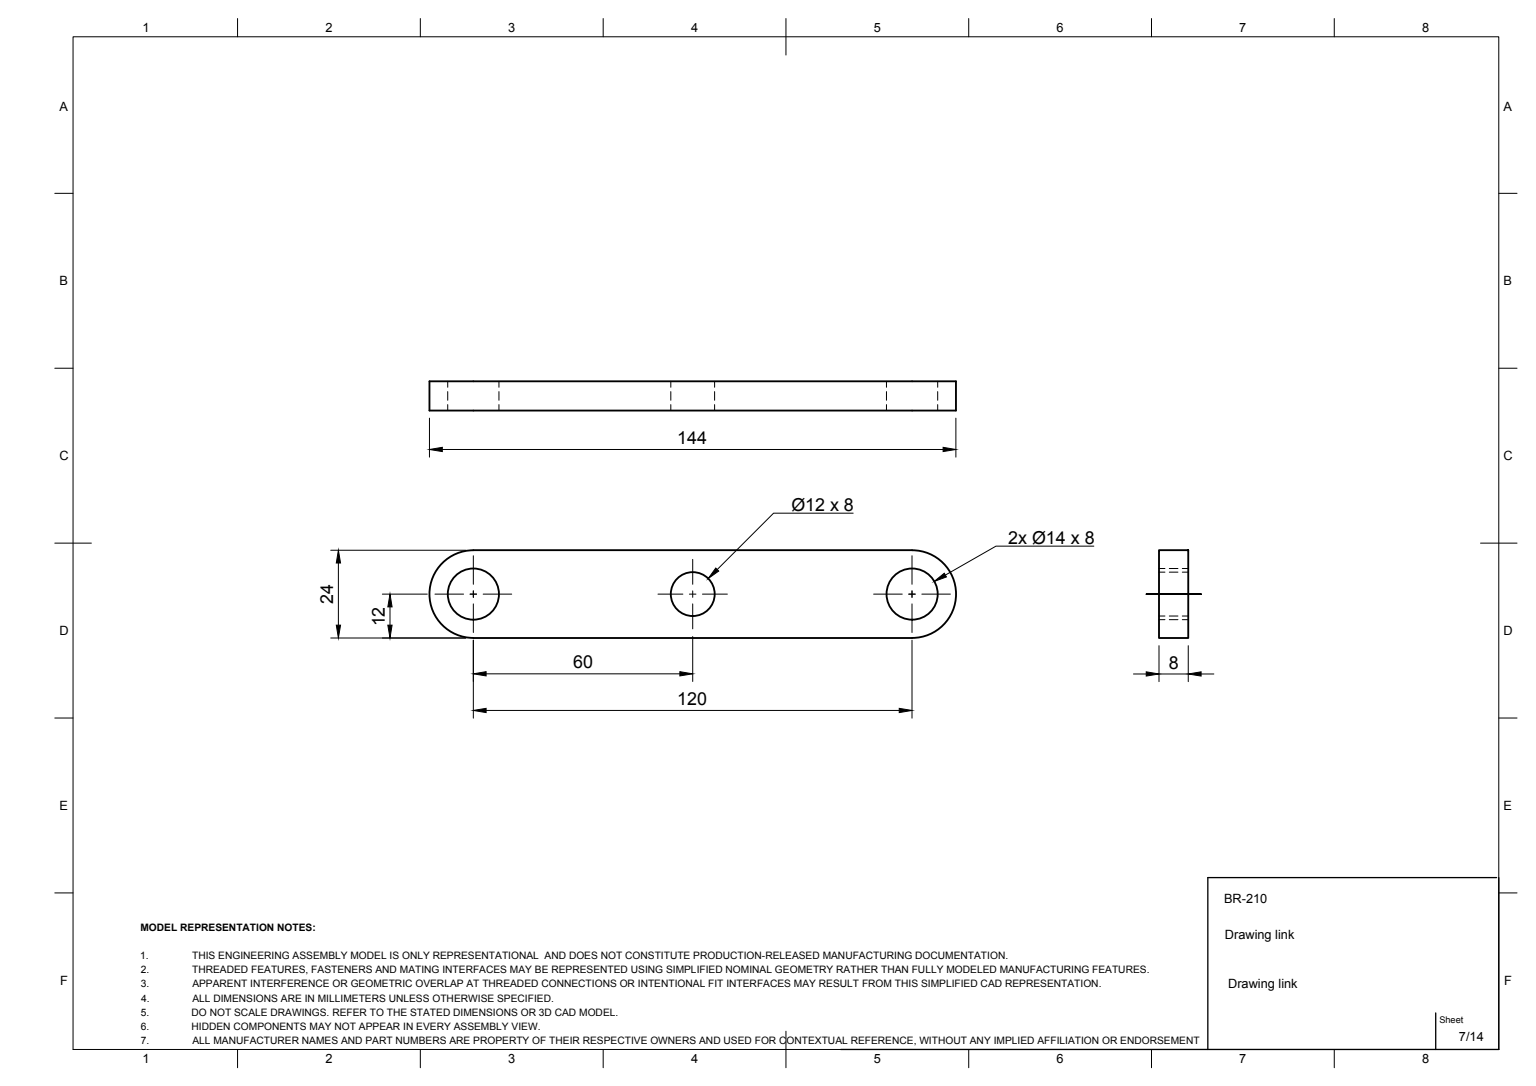
ISO-10303-21;
HEADER;
/* Generated by software containing ST-Developer
 * from STEP Tools, Inc. (www.steptools.com) 
 */

FILE_DESCRIPTION(
/* description */ ('Independent 1:2 reduction pantograph. 120 mm parallelogram sides; fix
ed fulcrum on the extension of a 240 mm link. Drawing point halfway al
ong its link, so its XY displacement is one half of the tracing point.
 Replaceable pivot bushes and retained pins. Calibration and productio
n accuracy unassigned.'),
/* implementation_level */ '2;1');

FILE_NAME(
/* name */ 'Drawing link.step',
/* time_stamp */ '2026-11-07T22:11:57-08:00',
/* author */ (''),
/* organization */ (''),
/* preprocessor_version */ 'ST-DEVELOPER v20.2',
/* originating_system */ 'Autodesk Translation Framework v15.17.0.0',
/* authorisation */ '');

FILE_SCHEMA (('AUTOMOTIVE_DESIGN { 1 0 10303 214 3 1 1 }'));
ENDSEC;

DATA;
#10=MECHANICAL_DESIGN_GEOMETRIC_PRESENTATION_REPRESENTATION('',(#189),#2926);
#163=SHAPE_REPRESENTATION_RELATIONSHIP('SRR','None',#3000,#176);
#176=ADVANCED_BREP_SHAPE_REPRESENTATION('',(#202),#2916);
#189=STYLED_ITEM('',(#3074),#202);
#202=MANIFOLD_SOLID_BREP('Body1',#1544);
#230=FACE_BOUND('',#447,.T.);
#231=FACE_BOUND('',#448,.T.);
#232=FACE_BOUND('',#449,.T.);
#233=FACE_BOUND('',#451,.T.);
#234=FACE_BOUND('',#452,.T.);
#235=FACE_BOUND('',#453,.T.);
#270=PLANE('',#1760);
#271=PLANE('',#1764);
#272=PLANE('',#1768);
#273=PLANE('',#1769);
#329=FACE_OUTER_BOUND('',#439,.T.);
#330=FACE_OUTER_BOUND('',#440,.T.);
#331=FACE_OUTER_BOUND('',#441,.T.);
#332=FACE_OUTER_BOUND('',#442,.T.);
#333=FACE_OUTER_BOUND('',#443,.T.);
#334=FACE_OUTER_BOUND('',#444,.T.);
#335=FACE_OUTER_BOUND('',#445,.T.);
#336=FACE_OUTER_BOUND('',#446,.T.);
#337=FACE_OUTER_BOUND('',#450,.T.);
#439=EDGE_LOOP('',(#1175,#1176,#1177,#1178));
#440=EDGE_LOOP('',(#1179,#1180,#1181,#1182));
#441=EDGE_LOOP('',(#1183,#1184,#1185,#1186));
#442=EDGE_LOOP('',(#1187,#1188,#1189,#1190));
#443=EDGE_LOOP('',(#1191,#1192,#1193,#1194));
#444=EDGE_LOOP('',(#1195,#1196,#1197,#1198));
#445=EDGE_LOOP('',(#1199,#1200,#1201,#1202));
#446=EDGE_LOOP('',(#1203,#1204,#1205,#1206));
#447=EDGE_LOOP('',(#1207));
#448=EDGE_LOOP('',(#1208));
#449=EDGE_LOOP('',(#1209));
#450=EDGE_LOOP('',(#1210,#1211,#1212,#1213));
#451=EDGE_LOOP('',(#1214));
#452=EDGE_LOOP('',(#1215));
#453=EDGE_LOOP('',(#1216));
#565=LINE('',#2595,#646);
#566=LINE('',#2601,#647);
#567=LINE('',#2607,#648);
#568=LINE('',#2612,#649);
#569=LINE('',#2614,#650);
#570=LINE('',#2616,#651);
#571=LINE('',#2617,#652);
#572=LINE('',#2623,#653);
#573=LINE('',#2626,#654);
#574=LINE('',#2628,#655);
#575=LINE('',#2629,#656);
#646=VECTOR('',#2069,6.);
#647=VECTOR('',#2076,7.);
#648=VECTOR('',#2083,7.);
#649=VECTOR('',#2088,10.);
#650=VECTOR('',#2089,10.);
#651=VECTOR('',#2090,10.);
#652=VECTOR('',#2091,10.);
#653=VECTOR('',#2098,10.);
#654=VECTOR('',#2101,10.);
#655=VECTOR('',#2102,10.);
#656=VECTOR('',#2103,10.);
#721=CIRCLE('',#1752,6.);
#722=CIRCLE('',#1753,6.);
#723=CIRCLE('',#1755,7.);
#724=CIRCLE('',#1756,7.);
#725=CIRCLE('',#1758,7.);
#726=CIRCLE('',#1759,7.);
#727=CIRCLE('',#1762,12.);
#728=CIRCLE('',#1763,12.);
#729=CIRCLE('',#1766,12.);
#730=CIRCLE('',#1767,12.);
#821=VERTEX_POINT('',#2592);
#822=VERTEX_POINT('',#2594);
#823=VERTEX_POINT('',#2598);
#824=VERTEX_POINT('',#2600);
#825=VERTEX_POINT('',#2604);
#826=VERTEX_POINT('',#2606);
#827=VERTEX_POINT('',#2610);
#828=VERTEX_POINT('',#2611);
#829=VERTEX_POINT('',#2613);
#830=VERTEX_POINT('',#2615);
#831=VERTEX_POINT('',#2619);
#832=VERTEX_POINT('',#2621);
#833=VERTEX_POINT('',#2625);
#834=VERTEX_POINT('',#2627);
#952=EDGE_CURVE('',#821,#821,#721,.T.);
#953=EDGE_CURVE('',#821,#822,#565,.T.);
#954=EDGE_CURVE('',#822,#822,#722,.T.);
#955=EDGE_CURVE('',#823,#823,#723,.T.);
#956=EDGE_CURVE('',#823,#824,#566,.T.);
#957=EDGE_CURVE('',#824,#824,#724,.T.);
#958=EDGE_CURVE('',#825,#825,#725,.T.);
#959=EDGE_CURVE('',#825,#826,#567,.T.);
#960=EDGE_CURVE('',#826,#826,#726,.T.);
#961=EDGE_CURVE('',#827,#828,#568,.T.);
#962=EDGE_CURVE('',#828,#829,#569,.T.);
#963=EDGE_CURVE('',#830,#829,#570,.T.);
#964=EDGE_CURVE('',#827,#830,#571,.T.);
#965=EDGE_CURVE('',#831,#827,#727,.T.);
#966=EDGE_CURVE('',#832,#830,#728,.T.);
#967=EDGE_CURVE('',#831,#832,#572,.T.);
#968=EDGE_CURVE('',#833,#831,#573,.T.);
#969=EDGE_CURVE('',#834,#832,#574,.T.);
#970=EDGE_CURVE('',#833,#834,#575,.T.);
#971=EDGE_CURVE('',#828,#833,#729,.T.);
#972=EDGE_CURVE('',#829,#834,#730,.T.);
#1175=ORIENTED_EDGE('',*,*,#952,.F.);
#1176=ORIENTED_EDGE('',*,*,#953,.T.);
#1177=ORIENTED_EDGE('',*,*,#954,.F.);
#1178=ORIENTED_EDGE('',*,*,#953,.F.);
#1179=ORIENTED_EDGE('',*,*,#955,.F.);
#1180=ORIENTED_EDGE('',*,*,#956,.T.);
#1181=ORIENTED_EDGE('',*,*,#957,.F.);
#1182=ORIENTED_EDGE('',*,*,#956,.F.);
#1183=ORIENTED_EDGE('',*,*,#958,.F.);
#1184=ORIENTED_EDGE('',*,*,#959,.T.);
#1185=ORIENTED_EDGE('',*,*,#960,.F.);
#1186=ORIENTED_EDGE('',*,*,#959,.F.);
#1187=ORIENTED_EDGE('',*,*,#961,.T.);
#1188=ORIENTED_EDGE('',*,*,#962,.T.);
#1189=ORIENTED_EDGE('',*,*,#963,.F.);
#1190=ORIENTED_EDGE('',*,*,#964,.F.);
#1191=ORIENTED_EDGE('',*,*,#965,.T.);
#1192=ORIENTED_EDGE('',*,*,#964,.T.);
#1193=ORIENTED_EDGE('',*,*,#966,.F.);
#1194=ORIENTED_EDGE('',*,*,#967,.F.);
#1195=ORIENTED_EDGE('',*,*,#968,.T.);
#1196=ORIENTED_EDGE('',*,*,#967,.T.);
#1197=ORIENTED_EDGE('',*,*,#969,.F.);
#1198=ORIENTED_EDGE('',*,*,#970,.F.);
#1199=ORIENTED_EDGE('',*,*,#971,.T.);
#1200=ORIENTED_EDGE('',*,*,#970,.T.);
#1201=ORIENTED_EDGE('',*,*,#972,.F.);
#1202=ORIENTED_EDGE('',*,*,#962,.F.);
#1203=ORIENTED_EDGE('',*,*,#972,.T.);
#1204=ORIENTED_EDGE('',*,*,#969,.T.);
#1205=ORIENTED_EDGE('',*,*,#966,.T.);
#1206=ORIENTED_EDGE('',*,*,#963,.T.);
#1207=ORIENTED_EDGE('',*,*,#952,.T.);
#1208=ORIENTED_EDGE('',*,*,#955,.T.);
#1209=ORIENTED_EDGE('',*,*,#958,.T.);
#1210=ORIENTED_EDGE('',*,*,#971,.F.);
#1211=ORIENTED_EDGE('',*,*,#961,.F.);
#1212=ORIENTED_EDGE('',*,*,#965,.F.);
#1213=ORIENTED_EDGE('',*,*,#968,.F.);
#1214=ORIENTED_EDGE('',*,*,#954,.T.);
#1215=ORIENTED_EDGE('',*,*,#957,.T.);
#1216=ORIENTED_EDGE('',*,*,#960,.T.);
#1417=CYLINDRICAL_SURFACE('',#1751,6.);
#1418=CYLINDRICAL_SURFACE('',#1754,7.);
#1419=CYLINDRICAL_SURFACE('',#1757,7.);
#1420=CYLINDRICAL_SURFACE('',#1761,12.);
#1421=CYLINDRICAL_SURFACE('',#1765,12.);
#1473=ADVANCED_FACE('',(#329),#1417,.F.);
#1474=ADVANCED_FACE('',(#330),#1418,.F.);
#1475=ADVANCED_FACE('',(#331),#1419,.F.);
#1476=ADVANCED_FACE('',(#332),#270,.T.);
#1477=ADVANCED_FACE('',(#333),#1420,.T.);
#1478=ADVANCED_FACE('',(#334),#271,.T.);
#1479=ADVANCED_FACE('',(#335),#1421,.T.);
#1480=ADVANCED_FACE('',(#336,#230,#231,#232),#272,.T.);
#1481=ADVANCED_FACE('',(#337,#233,#234,#235),#273,.F.);
#1544=CLOSED_SHELL('',(#1473,#1474,#1475,#1476,#1477,#1478,#1479,#1480,
#1481));
#1750=AXIS2_PLACEMENT_3D('',#2590,#2063,#2064);
#1751=AXIS2_PLACEMENT_3D('',#2591,#2065,#2066);
#1752=AXIS2_PLACEMENT_3D('',#2593,#2067,#2068);
#1753=AXIS2_PLACEMENT_3D('',#2596,#2070,#2071);
#1754=AXIS2_PLACEMENT_3D('',#2597,#2072,#2073);
#1755=AXIS2_PLACEMENT_3D('',#2599,#2074,#2075);
#1756=AXIS2_PLACEMENT_3D('',#2602,#2077,#2078);
#1757=AXIS2_PLACEMENT_3D('',#2603,#2079,#2080);
#1758=AXIS2_PLACEMENT_3D('',#2605,#2081,#2082);
#1759=AXIS2_PLACEMENT_3D('',#2608,#2084,#2085);
#1760=AXIS2_PLACEMENT_3D('',#2609,#2086,#2087);
#1761=AXIS2_PLACEMENT_3D('',#2618,#2092,#2093);
#1762=AXIS2_PLACEMENT_3D('',#2620,#2094,#2095);
#1763=AXIS2_PLACEMENT_3D('',#2622,#2096,#2097);
#1764=AXIS2_PLACEMENT_3D('',#2624,#2099,#2100);
#1765=AXIS2_PLACEMENT_3D('',#2630,#2104,#2105);
#1766=AXIS2_PLACEMENT_3D('',#2631,#2106,#2107);
#1767=AXIS2_PLACEMENT_3D('',#2632,#2108,#2109);
#1768=AXIS2_PLACEMENT_3D('',#2633,#2110,#2111);
#1769=AXIS2_PLACEMENT_3D('',#2634,#2112,#2113);
#2063=DIRECTION('axis',(0.,0.,1.));
#2064=DIRECTION('refdir',(1.,0.,0.));
#2065=DIRECTION('center_axis',(0.,0.,-1.));
#2066=DIRECTION('ref_axis',(1.,0.,0.));
#2067=DIRECTION('center_axis',(0.,0.,-1.));
#2068=DIRECTION('ref_axis',(1.,0.,0.));
#2069=DIRECTION('',(0.,0.,-1.));
#2070=DIRECTION('center_axis',(0.,0.,1.));
#2071=DIRECTION('ref_axis',(1.,0.,0.));
#2072=DIRECTION('center_axis',(0.,0.,-1.));
#2073=DIRECTION('ref_axis',(1.,0.,0.));
#2074=DIRECTION('center_axis',(0.,0.,-1.));
#2075=DIRECTION('ref_axis',(1.,0.,0.));
#2076=DIRECTION('',(0.,0.,-1.));
#2077=DIRECTION('center_axis',(0.,0.,1.));
#2078=DIRECTION('ref_axis',(1.,0.,0.));
#2079=DIRECTION('center_axis',(0.,0.,-1.));
#2080=DIRECTION('ref_axis',(1.,0.,0.));
#2081=DIRECTION('center_axis',(0.,0.,-1.));
#2082=DIRECTION('ref_axis',(1.,0.,0.));
#2083=DIRECTION('',(0.,0.,-1.));
#2084=DIRECTION('center_axis',(0.,0.,1.));
#2085=DIRECTION('ref_axis',(1.,0.,0.));
#2086=DIRECTION('center_axis',(0.,1.,0.));
#2087=DIRECTION('ref_axis',(-1.,0.,0.));
#2088=DIRECTION('',(-1.,0.,0.));
#2089=DIRECTION('',(0.,0.,1.));
#2090=DIRECTION('',(-1.,0.,0.));
#2091=DIRECTION('',(0.,0.,1.));
#2092=DIRECTION('center_axis',(0.,0.,1.));
#2093=DIRECTION('ref_axis',(0.,-1.,0.));
#2094=DIRECTION('center_axis',(0.,0.,1.));
#2095=DIRECTION('ref_axis',(0.,-1.,0.));
#2096=DIRECTION('center_axis',(0.,0.,1.));
#2097=DIRECTION('ref_axis',(0.,-1.,0.));
#2098=DIRECTION('',(0.,0.,1.));
#2099=DIRECTION('center_axis',(0.,-1.,0.));
#2100=DIRECTION('ref_axis',(1.,0.,0.));
#2101=DIRECTION('',(1.,0.,0.));
#2102=DIRECTION('',(1.,0.,0.));
#2103=DIRECTION('',(0.,0.,1.));
#2104=DIRECTION('center_axis',(0.,0.,1.));
#2105=DIRECTION('ref_axis',(0.,1.,0.));
#2106=DIRECTION('center_axis',(0.,0.,1.));
#2107=DIRECTION('ref_axis',(0.,1.,0.));
#2108=DIRECTION('center_axis',(0.,0.,1.));
#2109=DIRECTION('ref_axis',(0.,1.,0.));
#2110=DIRECTION('center_axis',(0.,0.,1.));
#2111=DIRECTION('ref_axis',(1.,0.,0.));
#2112=DIRECTION('center_axis',(0.,0.,1.));
#2113=DIRECTION('ref_axis',(1.,0.,0.));
#2590=CARTESIAN_POINT('',(0.,0.,0.));
#2591=CARTESIAN_POINT('Origin',(60.,0.,4.));
#2592=CARTESIAN_POINT('',(54.,7.34788079488412E-16,8.));
#2593=CARTESIAN_POINT('Origin',(60.,0.,8.));
#2594=CARTESIAN_POINT('',(54.,7.34788079488412E-16,0.));
#2595=CARTESIAN_POINT('',(54.,7.34788079488412E-16,4.));
#2596=CARTESIAN_POINT('Origin',(60.,0.,0.));
#2597=CARTESIAN_POINT('Origin',(0.,0.,4.));
#2598=CARTESIAN_POINT('',(-7.,8.57252759403147E-16,8.));
#2599=CARTESIAN_POINT('Origin',(0.,0.,8.));
#2600=CARTESIAN_POINT('',(-7.,8.57252759403147E-16,0.));
#2601=CARTESIAN_POINT('',(-7.,8.57252759403147E-16,4.));
#2602=CARTESIAN_POINT('Origin',(0.,0.,0.));
#2603=CARTESIAN_POINT('Origin',(120.,0.,4.));
#2604=CARTESIAN_POINT('',(113.,8.57252759403147E-16,8.));
#2605=CARTESIAN_POINT('Origin',(120.,0.,8.));
#2606=CARTESIAN_POINT('',(113.,8.57252759403147E-16,0.));
#2607=CARTESIAN_POINT('',(113.,8.57252759403147E-16,4.));
#2608=CARTESIAN_POINT('Origin',(120.,0.,0.));
#2609=CARTESIAN_POINT('Origin',(120.,12.,0.));
#2610=CARTESIAN_POINT('',(120.,12.,0.));
#2611=CARTESIAN_POINT('',(0.,12.,0.));
#2612=CARTESIAN_POINT('',(120.,12.,0.));
#2613=CARTESIAN_POINT('',(0.,12.,8.));
#2614=CARTESIAN_POINT('',(0.,12.,0.));
#2615=CARTESIAN_POINT('',(120.,12.,8.));
#2616=CARTESIAN_POINT('',(120.,12.,8.));
#2617=CARTESIAN_POINT('',(120.,12.,0.));
#2618=CARTESIAN_POINT('Origin',(120.,-1.11022302462516E-15,0.));
#2619=CARTESIAN_POINT('',(120.,-12.,0.));
#2620=CARTESIAN_POINT('Origin',(120.,-1.11022302462516E-15,0.));
#2621=CARTESIAN_POINT('',(120.,-12.,8.));
#2622=CARTESIAN_POINT('Origin',(120.,-1.11022302462516E-15,8.));
#2623=CARTESIAN_POINT('',(120.,-12.,0.));
#2624=CARTESIAN_POINT('Origin',(0.,-12.,0.));
#2625=CARTESIAN_POINT('',(-1.46957615897682E-15,-12.,0.));
#2626=CARTESIAN_POINT('',(0.,-12.,0.));
#2627=CARTESIAN_POINT('',(-1.46957615897682E-15,-12.,8.));
#2628=CARTESIAN_POINT('',(0.,-12.,8.));
#2629=CARTESIAN_POINT('',(-1.46957615897682E-15,-12.,0.));
#2630=CARTESIAN_POINT('Origin',(0.,0.,0.));
#2631=CARTESIAN_POINT('Origin',(0.,0.,0.));
#2632=CARTESIAN_POINT('Origin',(0.,0.,8.));
#2633=CARTESIAN_POINT('Origin',(60.,0.,8.));
#2634=CARTESIAN_POINT('Origin',(60.,0.,0.));
#2901=UNCERTAINTY_MEASURE_WITH_UNIT(LENGTH_MEASURE(0.01),#2927,
'DISTANCE_ACCURACY_VALUE',
'Maximum model space distance between geometric entities at asserted c
onnectivities');
#2911=UNCERTAINTY_MEASURE_WITH_UNIT(LENGTH_MEASURE(0.01),#2927,
'DISTANCE_ACCURACY_VALUE',
'Maximum model space distance between geometric entities at asserted c
onnectivities');
#2916=(
GEOMETRIC_REPRESENTATION_CONTEXT(3)
GLOBAL_UNCERTAINTY_ASSIGNED_CONTEXT((#2901))
GLOBAL_UNIT_ASSIGNED_CONTEXT((#2927,#2929,#2930))
REPRESENTATION_CONTEXT('','3D')
);
#2926=(
GEOMETRIC_REPRESENTATION_CONTEXT(3)
GLOBAL_UNCERTAINTY_ASSIGNED_CONTEXT((#2911))
GLOBAL_UNIT_ASSIGNED_CONTEXT((#2927,#2929,#2930))
REPRESENTATION_CONTEXT('','3D')
);
#2927=(
LENGTH_UNIT()
NAMED_UNIT(*)
SI_UNIT(.MILLI.,.METRE.)
);
#2929=(
NAMED_UNIT(*)
PLANE_ANGLE_UNIT()
SI_UNIT($,.RADIAN.)
);
#2930=(
NAMED_UNIT(*)
SI_UNIT($,.STERADIAN.)
SOLID_ANGLE_UNIT()
);
#2935=SHAPE_DEFINITION_REPRESENTATION(#2949,#3000);
#2949=PRODUCT_DEFINITION_SHAPE('',$,#3015);
#3000=SHAPE_REPRESENTATION('',(#1750),#2916);
#3010=PRODUCT_DEFINITION_CONTEXT('part definition',#3054,'design');
#3015=PRODUCT_DEFINITION('Drawing link','Drawing link',#3029,#3010);
#3029=PRODUCT_DEFINITION_FORMATION('',$,#3060);
#3054=APPLICATION_CONTEXT(
'Core Data for Automotive Mechanical Design Process');
#3055=PRODUCT_CONTEXT('part definition',#3054,'mechanical');
#3060=PRODUCT('Drawing link','Drawing link',$,(#3055));
#3074=PRESENTATION_STYLE_ASSIGNMENT((#3086));
#3086=SURFACE_STYLE_USAGE(.BOTH.,#3098);
#3098=SURFACE_SIDE_STYLE('',(#3110));
#3110=SURFACE_STYLE_FILL_AREA(#3122);
#3122=FILL_AREA_STYLE('Drawing link finish',(#3134));
#3134=FILL_AREA_STYLE_COLOUR('Drawing link finish',#3146);
#3146=COLOUR_RGB('Drawing link finish',0.662745098039216,0.831372549019608,
0.949019607843137);
ENDSEC;
END-ISO-10303-21;
